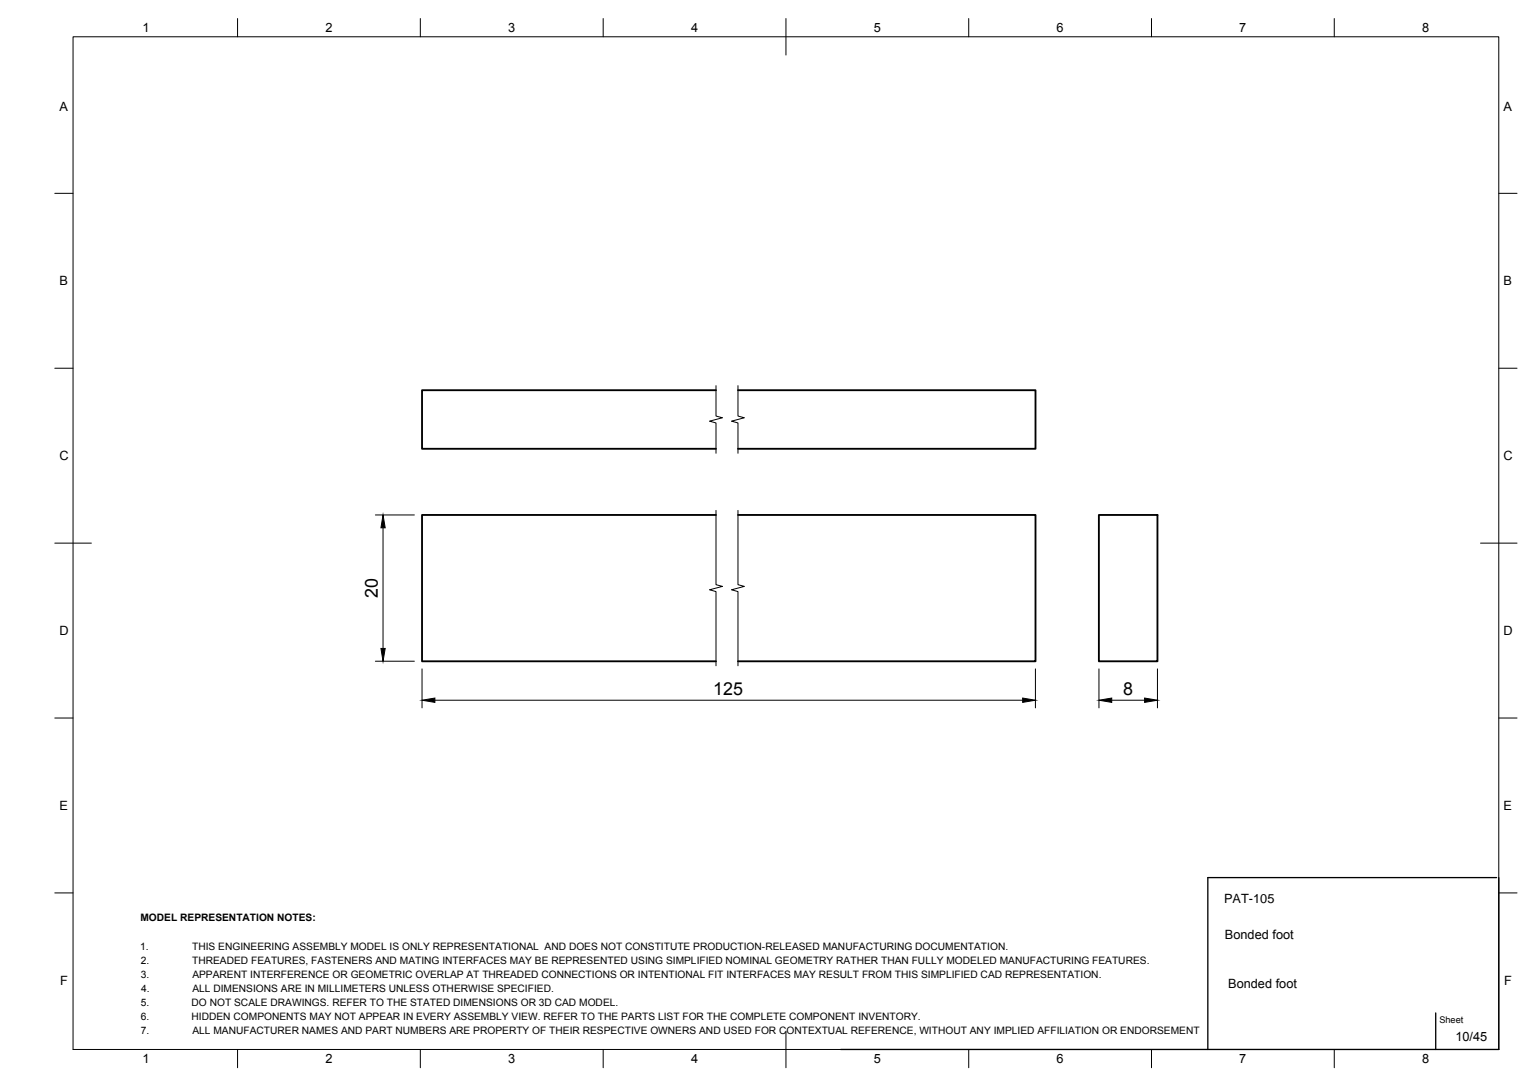
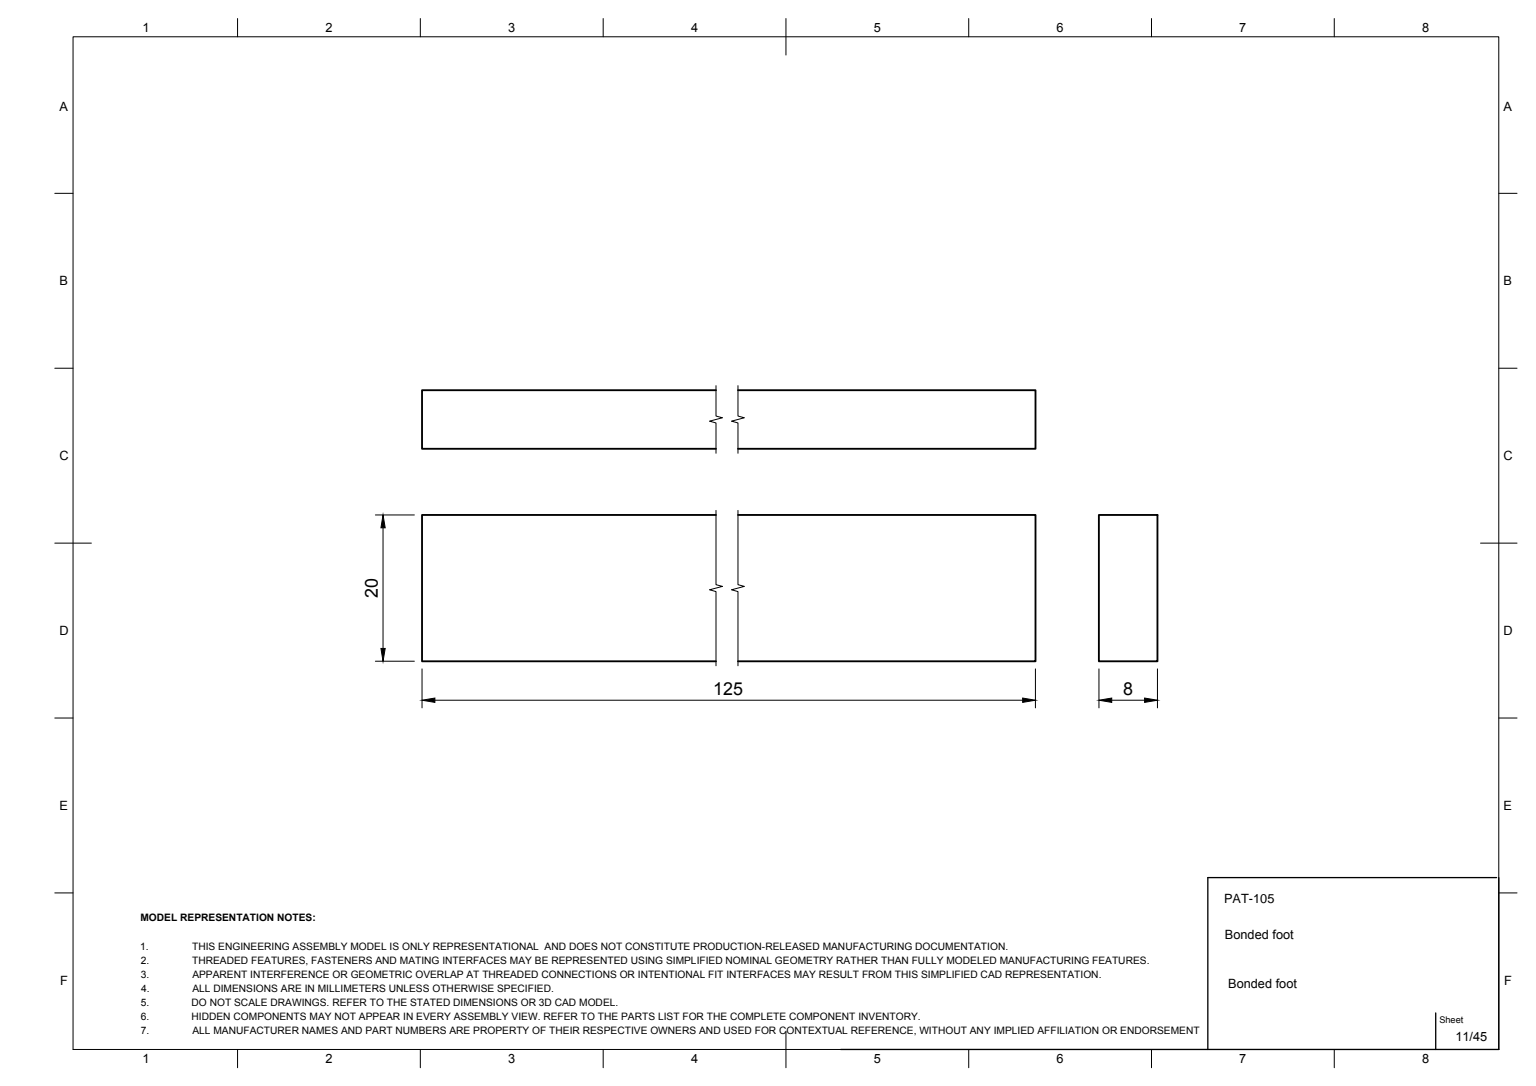
ISO-10303-21;
HEADER;
/* Generated by software containing ST-Developer
 * from STEP Tools, Inc. (www.steptools.com) 
 */

FILE_DESCRIPTION(
/* description */ ('Torque wrench calibration arm'),
/* implementation_level */ '2;1');

FILE_NAME(
/* name */ 'Bonded foot.step',
/* time_stamp */ '2026-10-28T03:24:52-07:00',
/* author */ (''),
/* organization */ (''),
/* preprocessor_version */ 'ST-DEVELOPER v20.2',
/* originating_system */ 'Autodesk Translation Framework v15.17.0.0',
/* authorisation */ '');

FILE_SCHEMA (('AUTOMOTIVE_DESIGN { 1 0 10303 214 3 1 1 }'));
ENDSEC;

DATA;
#10=MECHANICAL_DESIGN_GEOMETRIC_PRESENTATION_REPRESENTATION('',(#431),#12783);
#357=SHAPE_REPRESENTATION_RELATIONSHIP('SRR','None',#12938,#394);
#394=ADVANCED_BREP_SHAPE_REPRESENTATION('',(#485),#12747);
#431=STYLED_ITEM('',(#13226),#485);
#485=MANIFOLD_SOLID_BREP('Body1',#6500);
#698=PLANE('',#7144);
#699=PLANE('',#7145);
#700=PLANE('',#7146);
#701=PLANE('',#7147);
#702=PLANE('',#7148);
#703=PLANE('',#7149);
#963=FACE_OUTER_BOUND('',#1410,.T.);
#964=FACE_OUTER_BOUND('',#1411,.T.);
#965=FACE_OUTER_BOUND('',#1412,.T.);
#966=FACE_OUTER_BOUND('',#1413,.T.);
#967=FACE_OUTER_BOUND('',#1414,.T.);
#968=FACE_OUTER_BOUND('',#1415,.T.);
#1410=EDGE_LOOP('',(#4747,#4748,#4749,#4750));
#1411=EDGE_LOOP('',(#4751,#4752,#4753,#4754));
#1412=EDGE_LOOP('',(#4755,#4756,#4757,#4758));
#1413=EDGE_LOOP('',(#4759,#4760,#4761,#4762));
#1414=EDGE_LOOP('',(#4763,#4764,#4765,#4766));
#1415=EDGE_LOOP('',(#4767,#4768,#4769,#4770));
#1896=LINE('',#10354,#2311);
#1897=LINE('',#10356,#2312);
#1898=LINE('',#10358,#2313);
#1899=LINE('',#10359,#2314);
#1900=LINE('',#10362,#2315);
#1901=LINE('',#10364,#2316);
#1902=LINE('',#10365,#2317);
#1903=LINE('',#10368,#2318);
#1904=LINE('',#10370,#2319);
#1905=LINE('',#10371,#2320);
#1906=LINE('',#10373,#2321);
#1907=LINE('',#10374,#2322);
#2311=VECTOR('',#8290,1.);
#2312=VECTOR('',#8291,1.);
#2313=VECTOR('',#8292,1.);
#2314=VECTOR('',#8293,1.);
#2315=VECTOR('',#8296,1.);
#2316=VECTOR('',#8297,1.);
#2317=VECTOR('',#8298,1.);
#2318=VECTOR('',#8301,1.);
#2319=VECTOR('',#8302,1.);
#2320=VECTOR('',#8303,1.);
#2321=VECTOR('',#8306,1.);
#2322=VECTOR('',#8307,1.);
#3103=VERTEX_POINT('',#10352);
#3104=VERTEX_POINT('',#10353);
#3105=VERTEX_POINT('',#10355);
#3106=VERTEX_POINT('',#10357);
#3107=VERTEX_POINT('',#10361);
#3108=VERTEX_POINT('',#10363);
#3109=VERTEX_POINT('',#10367);
#3110=VERTEX_POINT('',#10369);
#3731=EDGE_CURVE('',#3103,#3104,#1896,.T.);
#3732=EDGE_CURVE('',#3104,#3105,#1897,.T.);
#3733=EDGE_CURVE('',#3106,#3105,#1898,.T.);
#3734=EDGE_CURVE('',#3103,#3106,#1899,.T.);
#3735=EDGE_CURVE('',#3107,#3103,#1900,.T.);
#3736=EDGE_CURVE('',#3108,#3106,#1901,.T.);
#3737=EDGE_CURVE('',#3107,#3108,#1902,.T.);
#3738=EDGE_CURVE('',#3109,#3107,#1903,.T.);
#3739=EDGE_CURVE('',#3110,#3108,#1904,.T.);
#3740=EDGE_CURVE('',#3109,#3110,#1905,.T.);
#3741=EDGE_CURVE('',#3104,#3109,#1906,.T.);
#3742=EDGE_CURVE('',#3105,#3110,#1907,.T.);
#4747=ORIENTED_EDGE('',*,*,#3731,.T.);
#4748=ORIENTED_EDGE('',*,*,#3732,.T.);
#4749=ORIENTED_EDGE('',*,*,#3733,.F.);
#4750=ORIENTED_EDGE('',*,*,#3734,.F.);
#4751=ORIENTED_EDGE('',*,*,#3735,.T.);
#4752=ORIENTED_EDGE('',*,*,#3734,.T.);
#4753=ORIENTED_EDGE('',*,*,#3736,.F.);
#4754=ORIENTED_EDGE('',*,*,#3737,.F.);
#4755=ORIENTED_EDGE('',*,*,#3738,.T.);
#4756=ORIENTED_EDGE('',*,*,#3737,.T.);
#4757=ORIENTED_EDGE('',*,*,#3739,.F.);
#4758=ORIENTED_EDGE('',*,*,#3740,.F.);
#4759=ORIENTED_EDGE('',*,*,#3741,.T.);
#4760=ORIENTED_EDGE('',*,*,#3740,.T.);
#4761=ORIENTED_EDGE('',*,*,#3742,.F.);
#4762=ORIENTED_EDGE('',*,*,#3732,.F.);
#4763=ORIENTED_EDGE('',*,*,#3742,.T.);
#4764=ORIENTED_EDGE('',*,*,#3739,.T.);
#4765=ORIENTED_EDGE('',*,*,#3736,.T.);
#4766=ORIENTED_EDGE('',*,*,#3733,.T.);
#4767=ORIENTED_EDGE('',*,*,#3741,.F.);
#4768=ORIENTED_EDGE('',*,*,#3731,.F.);
#4769=ORIENTED_EDGE('',*,*,#3735,.F.);
#4770=ORIENTED_EDGE('',*,*,#3738,.F.);
#6188=ADVANCED_FACE('',(#963),#698,.T.);
#6189=ADVANCED_FACE('',(#964),#699,.T.);
#6190=ADVANCED_FACE('',(#965),#700,.T.);
#6191=ADVANCED_FACE('',(#966),#701,.T.);
#6192=ADVANCED_FACE('',(#967),#702,.T.);
#6193=ADVANCED_FACE('',(#968),#703,.F.);
#6500=CLOSED_SHELL('',(#6188,#6189,#6190,#6191,#6192,#6193));
#7143=AXIS2_PLACEMENT_3D('',#10350,#8286,#8287);
#7144=AXIS2_PLACEMENT_3D('',#10351,#8288,#8289);
#7145=AXIS2_PLACEMENT_3D('',#10360,#8294,#8295);
#7146=AXIS2_PLACEMENT_3D('',#10366,#8299,#8300);
#7147=AXIS2_PLACEMENT_3D('',#10372,#8304,#8305);
#7148=AXIS2_PLACEMENT_3D('',#10375,#8308,#8309);
#7149=AXIS2_PLACEMENT_3D('',#10376,#8310,#8311);
#8286=DIRECTION('axis',(0.,0.,1.));
#8287=DIRECTION('refdir',(1.,0.,0.));
#8288=DIRECTION('center_axis',(0.,1.,0.));
#8289=DIRECTION('ref_axis',(-1.,0.,0.));
#8290=DIRECTION('',(-1.,0.,0.));
#8291=DIRECTION('',(0.,0.,1.));
#8292=DIRECTION('',(-1.,0.,0.));
#8293=DIRECTION('',(0.,0.,1.));
#8294=DIRECTION('center_axis',(1.,0.,0.));
#8295=DIRECTION('ref_axis',(0.,1.,0.));
#8296=DIRECTION('',(0.,1.,0.));
#8297=DIRECTION('',(0.,1.,0.));
#8298=DIRECTION('',(0.,0.,1.));
#8299=DIRECTION('center_axis',(0.,-1.,0.));
#8300=DIRECTION('ref_axis',(1.,0.,0.));
#8301=DIRECTION('',(1.,0.,0.));
#8302=DIRECTION('',(1.,0.,0.));
#8303=DIRECTION('',(0.,0.,1.));
#8304=DIRECTION('center_axis',(-1.,0.,0.));
#8305=DIRECTION('ref_axis',(0.,-1.,0.));
#8306=DIRECTION('',(0.,-1.,0.));
#8307=DIRECTION('',(0.,-1.,0.));
#8308=DIRECTION('center_axis',(0.,0.,1.));
#8309=DIRECTION('ref_axis',(1.,0.,0.));
#8310=DIRECTION('center_axis',(0.,0.,1.));
#8311=DIRECTION('ref_axis',(1.,0.,0.));
#10350=CARTESIAN_POINT('',(0.,0.,0.));
#10351=CARTESIAN_POINT('Origin',(-4.,10.5,-0.8));
#10352=CARTESIAN_POINT('',(-4.,10.5,-0.8));
#10353=CARTESIAN_POINT('',(-6.,10.5,-0.8));
#10354=CARTESIAN_POINT('',(-4.,10.5,-0.8));
#10355=CARTESIAN_POINT('',(-6.,10.5,0.));
#10356=CARTESIAN_POINT('',(-6.,10.5,-0.8));
#10357=CARTESIAN_POINT('',(-4.,10.5,0.));
#10358=CARTESIAN_POINT('',(-4.,10.5,0.));
#10359=CARTESIAN_POINT('',(-4.,10.5,-0.8));
#10360=CARTESIAN_POINT('Origin',(-4.,-2.,-0.8));
#10361=CARTESIAN_POINT('',(-4.,-2.,-0.8));
#10362=CARTESIAN_POINT('',(-4.,-2.,-0.8));
#10363=CARTESIAN_POINT('',(-4.,-2.,0.));
#10364=CARTESIAN_POINT('',(-4.,-2.,0.));
#10365=CARTESIAN_POINT('',(-4.,-2.,-0.8));
#10366=CARTESIAN_POINT('Origin',(-6.,-2.,-0.8));
#10367=CARTESIAN_POINT('',(-6.,-2.,-0.8));
#10368=CARTESIAN_POINT('',(-6.,-2.,-0.8));
#10369=CARTESIAN_POINT('',(-6.,-2.,0.));
#10370=CARTESIAN_POINT('',(-6.,-2.,0.));
#10371=CARTESIAN_POINT('',(-6.,-2.,-0.8));
#10372=CARTESIAN_POINT('Origin',(-6.,10.5,-0.8));
#10373=CARTESIAN_POINT('',(-6.,10.5,-0.8));
#10374=CARTESIAN_POINT('',(-6.,10.5,0.));
#10375=CARTESIAN_POINT('Origin',(-5.,4.25,0.));
#10376=CARTESIAN_POINT('Origin',(-5.,4.25,-0.8));
#12703=UNCERTAINTY_MEASURE_WITH_UNIT(LENGTH_MEASURE(0.001),#12784,
'DISTANCE_ACCURACY_VALUE',
'Maximum model space distance between geometric entities at asserted c
onnectivities');
#12739=UNCERTAINTY_MEASURE_WITH_UNIT(LENGTH_MEASURE(0.001),#12784,
'DISTANCE_ACCURACY_VALUE',
'Maximum model space distance between geometric entities at asserted c
onnectivities');
#12747=(
GEOMETRIC_REPRESENTATION_CONTEXT(3)
GLOBAL_UNCERTAINTY_ASSIGNED_CONTEXT((#12703))
GLOBAL_UNIT_ASSIGNED_CONTEXT((#12784,#12786,#12787))
REPRESENTATION_CONTEXT('','3D')
);
#12783=(
GEOMETRIC_REPRESENTATION_CONTEXT(3)
GLOBAL_UNCERTAINTY_ASSIGNED_CONTEXT((#12739))
GLOBAL_UNIT_ASSIGNED_CONTEXT((#12784,#12786,#12787))
REPRESENTATION_CONTEXT('','3D')
);
#12784=(
LENGTH_UNIT()
NAMED_UNIT(*)
SI_UNIT(.CENTI.,.METRE.)
);
#12786=(
NAMED_UNIT(*)
PLANE_ANGLE_UNIT()
SI_UNIT($,.RADIAN.)
);
#12787=(
NAMED_UNIT(*)
SI_UNIT($,.STERADIAN.)
SOLID_ANGLE_UNIT()
);
#12795=SHAPE_DEFINITION_REPRESENTATION(#12838,#12938);
#12838=PRODUCT_DEFINITION_SHAPE('',$,#12982);
#12938=SHAPE_REPRESENTATION('',(#7143),#12747);
#12974=PRODUCT_DEFINITION_CONTEXT('part definition',#13105,'design');
#12982=PRODUCT_DEFINITION('Bonded foot','Bonded foot',#13025,#12974);
#13025=PRODUCT_DEFINITION_FORMATION('',$,#13114);
#13105=APPLICATION_CONTEXT(
'Core Data for Automotive Mechanical Design Process');
#13106=PRODUCT_CONTEXT('part definition',#13105,'mechanical');
#13114=PRODUCT('Bonded foot','Bonded foot','Bonded foot',(#13106));
#13220=COLOUR_RGB('Off White',0.89,0.88,0.83);
#13221=FILL_AREA_STYLE_COLOUR('',#13220);
#13222=FILL_AREA_STYLE('',(#13221));
#13223=SURFACE_STYLE_FILL_AREA(#13222);
#13224=SURFACE_SIDE_STYLE('',(#13223));
#13225=SURFACE_STYLE_USAGE(.BOTH.,#13224);
#13226=PRESENTATION_STYLE_ASSIGNMENT((#13225));
ENDSEC;
END-ISO-10303-21;
